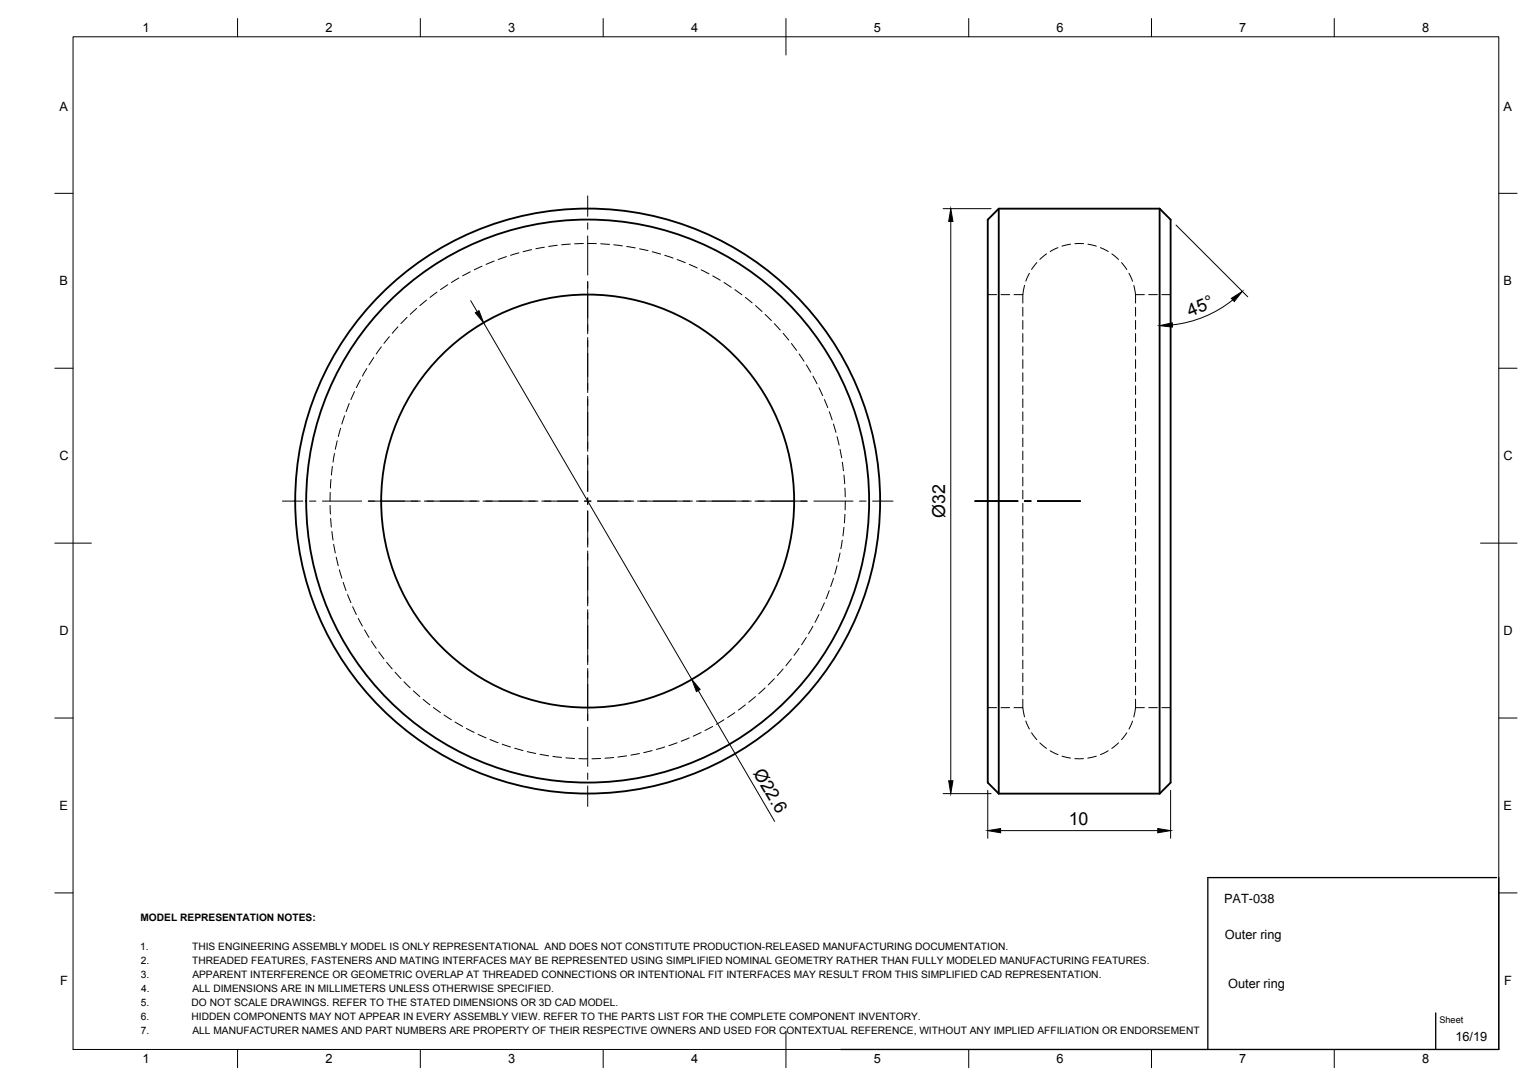
ISO-10303-21;
HEADER;
/* Generated by software containing ST-Developer
 * from STEP Tools, Inc. (www.steptools.com) 
 */

FILE_DESCRIPTION(
/* description */ ('Fork-mounted skate wheel'),
/* implementation_level */ '2;1');

FILE_NAME(
/* name */ 'Outer ring.step',
/* time_stamp */ '2026-10-29T16:11:26-07:00',
/* author */ (''),
/* organization */ (''),
/* preprocessor_version */ 'ST-DEVELOPER v20.2',
/* originating_system */ 'Autodesk Translation Framework v15.17.0.0',
/* authorisation */ '');

FILE_SCHEMA (('AUTOMOTIVE_DESIGN { 1 0 10303 214 3 1 1 }'));
ENDSEC;

DATA;
#10=MECHANICAL_DESIGN_GEOMETRIC_PRESENTATION_REPRESENTATION('',(#153),#3688);
#40=TOROIDAL_SURFACE('',#2099,1.1,0.309556);
#118=CONICAL_SURFACE('',#2110,1.57,0.785398163397449);
#119=CONICAL_SURFACE('',#2114,1.57,0.785398163397449);
#129=SHAPE_REPRESENTATION_RELATIONSHIP('SRR','None',#3754,#141);
#141=ADVANCED_BREP_SHAPE_REPRESENTATION('',(#171),#3683);
#153=STYLED_ITEM('',(#3896),#171);
#171=MANIFOLD_SOLID_BREP('Body1',#1815);
#210=FACE_BOUND('',#488,.T.);
#211=FACE_BOUND('',#493,.T.);
#260=PLANE('',#2107);
#261=PLANE('',#2116);
#345=FACE_OUTER_BOUND('',#485,.T.);
#346=FACE_OUTER_BOUND('',#486,.T.);
#347=FACE_OUTER_BOUND('',#487,.T.);
#348=FACE_OUTER_BOUND('',#489,.T.);
#349=FACE_OUTER_BOUND('',#490,.T.);
#350=FACE_OUTER_BOUND('',#491,.T.);
#351=FACE_OUTER_BOUND('',#492,.T.);
#352=FACE_OUTER_BOUND('',#494,.T.);
#485=EDGE_LOOP('',(#1483,#1484,#1485,#1486,#1487,#1488));
#486=EDGE_LOOP('',(#1489,#1490,#1491,#1492,#1493));
#487=EDGE_LOOP('',(#1494));
#488=EDGE_LOOP('',(#1495));
#489=EDGE_LOOP('',(#1496,#1497,#1498,#1499));
#490=EDGE_LOOP('',(#1500,#1501,#1502,#1503));
#491=EDGE_LOOP('',(#1504,#1505,#1506,#1507));
#492=EDGE_LOOP('',(#1508));
#493=EDGE_LOOP('',(#1509));
#494=EDGE_LOOP('',(#1510,#1511,#1512,#1513,#1514));
#619=LINE('',#3157,#713);
#620=LINE('',#3166,#714);
#621=LINE('',#3170,#715);
#622=LINE('',#3174,#716);
#623=LINE('',#3177,#717);
#713=VECTOR('',#2596,1.129765);
#714=VECTOR('',#2607,1.57);
#715=VECTOR('',#2612,1.6);
#716=VECTOR('',#2617,1.57);
#717=VECTOR('',#2622,1.129765);
#778=CIRCLE('',#2100,1.129765);
#779=CIRCLE('',#2101,1.129765);
#780=CIRCLE('',#2102,0.309556);
#781=CIRCLE('',#2103,1.129765);
#782=CIRCLE('',#2104,1.129765);
#783=CIRCLE('',#2106,1.129765);
#784=CIRCLE('',#2108,1.54);
#785=CIRCLE('',#2109,1.129765);
#786=CIRCLE('',#2111,1.6);
#787=CIRCLE('',#2113,1.6);
#788=CIRCLE('',#2115,1.54);
#927=VERTEX_POINT('',#3145);
#928=VERTEX_POINT('',#3146);
#929=VERTEX_POINT('',#3149);
#930=VERTEX_POINT('',#3151);
#931=VERTEX_POINT('',#3155);
#932=VERTEX_POINT('',#3159);
#933=VERTEX_POINT('',#3161);
#934=VERTEX_POINT('',#3164);
#935=VERTEX_POINT('',#3168);
#936=VERTEX_POINT('',#3172);
#1128=EDGE_CURVE('',#927,#928,#778,.T.);
#1129=EDGE_CURVE('',#928,#927,#779,.T.);
#1130=EDGE_CURVE('',#928,#929,#780,.T.);
#1131=EDGE_CURVE('',#930,#929,#781,.T.);
#1132=EDGE_CURVE('',#929,#930,#782,.T.);
#1133=EDGE_CURVE('',#931,#931,#783,.T.);
#1134=EDGE_CURVE('',#931,#930,#619,.T.);
#1135=EDGE_CURVE('',#932,#932,#784,.T.);
#1136=EDGE_CURVE('',#933,#933,#785,.T.);
#1137=EDGE_CURVE('',#934,#934,#786,.T.);
#1138=EDGE_CURVE('',#934,#932,#620,.T.);
#1139=EDGE_CURVE('',#935,#935,#787,.T.);
#1140=EDGE_CURVE('',#935,#934,#621,.T.);
#1141=EDGE_CURVE('',#936,#936,#788,.T.);
#1142=EDGE_CURVE('',#936,#935,#622,.T.);
#1143=EDGE_CURVE('',#927,#933,#623,.T.);
#1483=ORIENTED_EDGE('',*,*,#1128,.F.);
#1484=ORIENTED_EDGE('',*,*,#1129,.F.);
#1485=ORIENTED_EDGE('',*,*,#1130,.T.);
#1486=ORIENTED_EDGE('',*,*,#1131,.F.);
#1487=ORIENTED_EDGE('',*,*,#1132,.F.);
#1488=ORIENTED_EDGE('',*,*,#1130,.F.);
#1489=ORIENTED_EDGE('',*,*,#1133,.T.);
#1490=ORIENTED_EDGE('',*,*,#1134,.T.);
#1491=ORIENTED_EDGE('',*,*,#1131,.T.);
#1492=ORIENTED_EDGE('',*,*,#1132,.T.);
#1493=ORIENTED_EDGE('',*,*,#1134,.F.);
#1494=ORIENTED_EDGE('',*,*,#1135,.F.);
#1495=ORIENTED_EDGE('',*,*,#1136,.T.);
#1496=ORIENTED_EDGE('',*,*,#1137,.F.);
#1497=ORIENTED_EDGE('',*,*,#1138,.T.);
#1498=ORIENTED_EDGE('',*,*,#1135,.T.);
#1499=ORIENTED_EDGE('',*,*,#1138,.F.);
#1500=ORIENTED_EDGE('',*,*,#1139,.F.);
#1501=ORIENTED_EDGE('',*,*,#1140,.T.);
#1502=ORIENTED_EDGE('',*,*,#1137,.T.);
#1503=ORIENTED_EDGE('',*,*,#1140,.F.);
#1504=ORIENTED_EDGE('',*,*,#1141,.F.);
#1505=ORIENTED_EDGE('',*,*,#1142,.T.);
#1506=ORIENTED_EDGE('',*,*,#1139,.T.);
#1507=ORIENTED_EDGE('',*,*,#1142,.F.);
#1508=ORIENTED_EDGE('',*,*,#1141,.T.);
#1509=ORIENTED_EDGE('',*,*,#1133,.F.);
#1510=ORIENTED_EDGE('',*,*,#1128,.T.);
#1511=ORIENTED_EDGE('',*,*,#1129,.T.);
#1512=ORIENTED_EDGE('',*,*,#1143,.T.);
#1513=ORIENTED_EDGE('',*,*,#1136,.F.);
#1514=ORIENTED_EDGE('',*,*,#1143,.F.);
#1683=CYLINDRICAL_SURFACE('',#2105,1.129765);
#1684=CYLINDRICAL_SURFACE('',#2112,1.6);
#1685=CYLINDRICAL_SURFACE('',#2117,1.129765);
#1763=ADVANCED_FACE('',(#345),#40,.F.);
#1764=ADVANCED_FACE('',(#346),#1683,.F.);
#1765=ADVANCED_FACE('',(#347,#210),#260,.T.);
#1766=ADVANCED_FACE('',(#348),#118,.T.);
#1767=ADVANCED_FACE('',(#349),#1684,.T.);
#1768=ADVANCED_FACE('',(#350),#119,.T.);
#1769=ADVANCED_FACE('',(#351,#211),#261,.T.);
#1770=ADVANCED_FACE('',(#352),#1685,.F.);
#1815=CLOSED_SHELL('',(#1763,#1764,#1765,#1766,#1767,#1768,#1769,#1770));
#2098=AXIS2_PLACEMENT_3D('',#3143,#2578,#2579);
#2099=AXIS2_PLACEMENT_3D('',#3144,#2580,#2581);
#2100=AXIS2_PLACEMENT_3D('',#3147,#2582,#2583);
#2101=AXIS2_PLACEMENT_3D('',#3148,#2584,#2585);
#2102=AXIS2_PLACEMENT_3D('',#3150,#2586,#2587);
#2103=AXIS2_PLACEMENT_3D('',#3152,#2588,#2589);
#2104=AXIS2_PLACEMENT_3D('',#3153,#2590,#2591);
#2105=AXIS2_PLACEMENT_3D('',#3154,#2592,#2593);
#2106=AXIS2_PLACEMENT_3D('',#3156,#2594,#2595);
#2107=AXIS2_PLACEMENT_3D('',#3158,#2597,#2598);
#2108=AXIS2_PLACEMENT_3D('',#3160,#2599,#2600);
#2109=AXIS2_PLACEMENT_3D('',#3162,#2601,#2602);
#2110=AXIS2_PLACEMENT_3D('',#3163,#2603,#2604);
#2111=AXIS2_PLACEMENT_3D('',#3165,#2605,#2606);
#2112=AXIS2_PLACEMENT_3D('',#3167,#2608,#2609);
#2113=AXIS2_PLACEMENT_3D('',#3169,#2610,#2611);
#2114=AXIS2_PLACEMENT_3D('',#3171,#2613,#2614);
#2115=AXIS2_PLACEMENT_3D('',#3173,#2615,#2616);
#2116=AXIS2_PLACEMENT_3D('',#3175,#2618,#2619);
#2117=AXIS2_PLACEMENT_3D('',#3176,#2620,#2621);
#2578=DIRECTION('axis',(0.,0.,1.));
#2579=DIRECTION('refdir',(1.,0.,0.));
#2580=DIRECTION('center_axis',(0.,-1.,0.));
#2581=DIRECTION('ref_axis',(0.,0.,-1.));
#2582=DIRECTION('center_axis',(0.,-1.,0.));
#2583=DIRECTION('ref_axis',(1.,0.,0.));
#2584=DIRECTION('center_axis',(0.,-1.,0.));
#2585=DIRECTION('ref_axis',(1.,0.,0.));
#2586=DIRECTION('center_axis',(1.,0.,1.22464679914735E-16));
#2587=DIRECTION('ref_axis',(-1.22464679914735E-16,0.,1.));
#2588=DIRECTION('center_axis',(0.,1.,0.));
#2589=DIRECTION('ref_axis',(1.,0.,0.));
#2590=DIRECTION('center_axis',(0.,1.,0.));
#2591=DIRECTION('ref_axis',(1.,0.,0.));
#2592=DIRECTION('center_axis',(0.,-1.,0.));
#2593=DIRECTION('ref_axis',(1.,0.,0.));
#2594=DIRECTION('center_axis',(0.,-1.,0.));
#2595=DIRECTION('ref_axis',(1.,0.,0.));
#2596=DIRECTION('',(0.,1.,0.));
#2597=DIRECTION('center_axis',(0.,1.,0.));
#2598=DIRECTION('ref_axis',(0.,0.,1.));
#2599=DIRECTION('center_axis',(0.,-1.,0.));
#2600=DIRECTION('ref_axis',(1.,0.,0.));
#2601=DIRECTION('center_axis',(0.,-1.,0.));
#2602=DIRECTION('ref_axis',(1.,0.,0.));
#2603=DIRECTION('center_axis',(0.,-1.,0.));
#2604=DIRECTION('ref_axis',(1.,0.,0.));
#2605=DIRECTION('center_axis',(0.,-1.,0.));
#2606=DIRECTION('ref_axis',(1.,0.,0.));
#2607=DIRECTION('',(0.707106781186548,0.707106781186547,8.65956056235494E-17));
#2608=DIRECTION('center_axis',(0.,-1.,0.));
#2609=DIRECTION('ref_axis',(1.,0.,0.));
#2610=DIRECTION('center_axis',(0.,-1.,0.));
#2611=DIRECTION('ref_axis',(1.,0.,0.));
#2612=DIRECTION('',(0.,1.,0.));
#2613=DIRECTION('center_axis',(0.,1.,0.));
#2614=DIRECTION('ref_axis',(1.,0.,0.));
#2615=DIRECTION('center_axis',(0.,-1.,0.));
#2616=DIRECTION('ref_axis',(1.,0.,0.));
#2617=DIRECTION('',(-0.707106781186548,0.707106781186547,-8.65956056235494E-17));
#2618=DIRECTION('center_axis',(0.,-1.,0.));
#2619=DIRECTION('ref_axis',(0.,0.,-1.));
#2620=DIRECTION('center_axis',(0.,-1.,0.));
#2621=DIRECTION('ref_axis',(1.,0.,0.));
#2622=DIRECTION('',(0.,1.,0.));
#3143=CARTESIAN_POINT('',(0.,0.,0.));
#3144=CARTESIAN_POINT('Origin',(0.,0.,0.));
#3145=CARTESIAN_POINT('',(-1.129765,0.308121667383195,-1.38356309103871E-16));
#3146=CARTESIAN_POINT('',(-1.38356309103871E-16,0.308121667383195,1.129765));
#3147=CARTESIAN_POINT('Origin',(0.,0.308121667383195,0.));
#3148=CARTESIAN_POINT('Origin',(0.,0.308121667383195,0.));
#3149=CARTESIAN_POINT('',(-1.38356309103871E-16,-0.308121667383195,1.129765));
#3150=CARTESIAN_POINT('Origin',(-1.34711147906209E-16,0.,1.1));
#3151=CARTESIAN_POINT('',(-1.129765,-0.308121667383195,1.38356309103871E-16));
#3152=CARTESIAN_POINT('Origin',(0.,-0.308121667383195,0.));
#3153=CARTESIAN_POINT('Origin',(0.,-0.308121667383195,0.));
#3154=CARTESIAN_POINT('Origin',(0.,0.,0.));
#3155=CARTESIAN_POINT('',(-1.129765,-0.5,-1.38356309103871E-16));
#3156=CARTESIAN_POINT('Origin',(0.,-0.5,0.));
#3157=CARTESIAN_POINT('',(-1.129765,0.,-1.38356309103871E-16));
#3158=CARTESIAN_POINT('Origin',(1.54,0.5,0.));
#3159=CARTESIAN_POINT('',(-1.54,0.5,-1.88595607068692E-16));
#3160=CARTESIAN_POINT('Origin',(0.,0.5,0.));
#3161=CARTESIAN_POINT('',(-1.129765,0.5,-1.38356309103871E-16));
#3162=CARTESIAN_POINT('Origin',(0.,0.5,0.));
#3163=CARTESIAN_POINT('Origin',(0.,0.47,0.));
#3164=CARTESIAN_POINT('',(-1.6,0.44,-1.95943487863577E-16));
#3165=CARTESIAN_POINT('Origin',(0.,0.44,0.));
#3166=CARTESIAN_POINT('',(-1.57,0.47,-1.92269547466134E-16));
#3167=CARTESIAN_POINT('Origin',(0.,0.,0.));
#3168=CARTESIAN_POINT('',(-1.6,-0.44,-1.95943487863577E-16));
#3169=CARTESIAN_POINT('Origin',(0.,-0.44,0.));
#3170=CARTESIAN_POINT('',(-1.6,0.,-1.95943487863577E-16));
#3171=CARTESIAN_POINT('Origin',(0.,-0.47,0.));
#3172=CARTESIAN_POINT('',(-1.54,-0.5,-1.88595607068692E-16));
#3173=CARTESIAN_POINT('Origin',(0.,-0.5,0.));
#3174=CARTESIAN_POINT('',(-1.57,-0.47,-1.92269547466134E-16));
#3175=CARTESIAN_POINT('Origin',(1.129765,-0.5,0.));
#3176=CARTESIAN_POINT('Origin',(0.,0.,0.));
#3177=CARTESIAN_POINT('',(-1.129765,0.,-1.38356309103871E-16));
#3666=UNCERTAINTY_MEASURE_WITH_UNIT(LENGTH_MEASURE(0.001),#3689,
'DISTANCE_ACCURACY_VALUE',
'Maximum model space distance between geometric entities at asserted c
onnectivities');
#3671=UNCERTAINTY_MEASURE_WITH_UNIT(LENGTH_MEASURE(0.001),#3689,
'DISTANCE_ACCURACY_VALUE',
'Maximum model space distance between geometric entities at asserted c
onnectivities');
#3683=(
GEOMETRIC_REPRESENTATION_CONTEXT(3)
GLOBAL_UNCERTAINTY_ASSIGNED_CONTEXT((#3666))
GLOBAL_UNIT_ASSIGNED_CONTEXT((#3689,#3691,#3692))
REPRESENTATION_CONTEXT('','3D')
);
#3688=(
GEOMETRIC_REPRESENTATION_CONTEXT(3)
GLOBAL_UNCERTAINTY_ASSIGNED_CONTEXT((#3671))
GLOBAL_UNIT_ASSIGNED_CONTEXT((#3689,#3691,#3692))
REPRESENTATION_CONTEXT('','3D')
);
#3689=(
LENGTH_UNIT()
NAMED_UNIT(*)
SI_UNIT(.CENTI.,.METRE.)
);
#3691=(
NAMED_UNIT(*)
PLANE_ANGLE_UNIT()
SI_UNIT($,.RADIAN.)
);
#3692=(
NAMED_UNIT(*)
SI_UNIT($,.STERADIAN.)
SOLID_ANGLE_UNIT()
);
#3704=SHAPE_DEFINITION_REPRESENTATION(#3726,#3754);
#3726=PRODUCT_DEFINITION_SHAPE('',$,#3771);
#3754=SHAPE_REPRESENTATION('',(#2098),#3683);
#3759=PRODUCT_DEFINITION_CONTEXT('part definition',#3809,'design');
#3771=PRODUCT_DEFINITION('Outer ring','Outer ring',#3787,#3759);
#3787=PRODUCT_DEFINITION_FORMATION('',$,#3822);
#3809=APPLICATION_CONTEXT(
'Core Data for Automotive Mechanical Design Process');
#3810=PRODUCT_CONTEXT('part definition',#3809,'mechanical');
#3822=PRODUCT('Outer ring','Outer ring','Outer ring',(#3810));
#3890=COLOUR_RGB('Grey',0.48,0.52,0.57);
#3891=FILL_AREA_STYLE_COLOUR('',#3890);
#3892=FILL_AREA_STYLE('',(#3891));
#3893=SURFACE_STYLE_FILL_AREA(#3892);
#3894=SURFACE_SIDE_STYLE('',(#3893));
#3895=SURFACE_STYLE_USAGE(.BOTH.,#3894);
#3896=PRESENTATION_STYLE_ASSIGNMENT((#3895));
ENDSEC;
END-ISO-10303-21;
